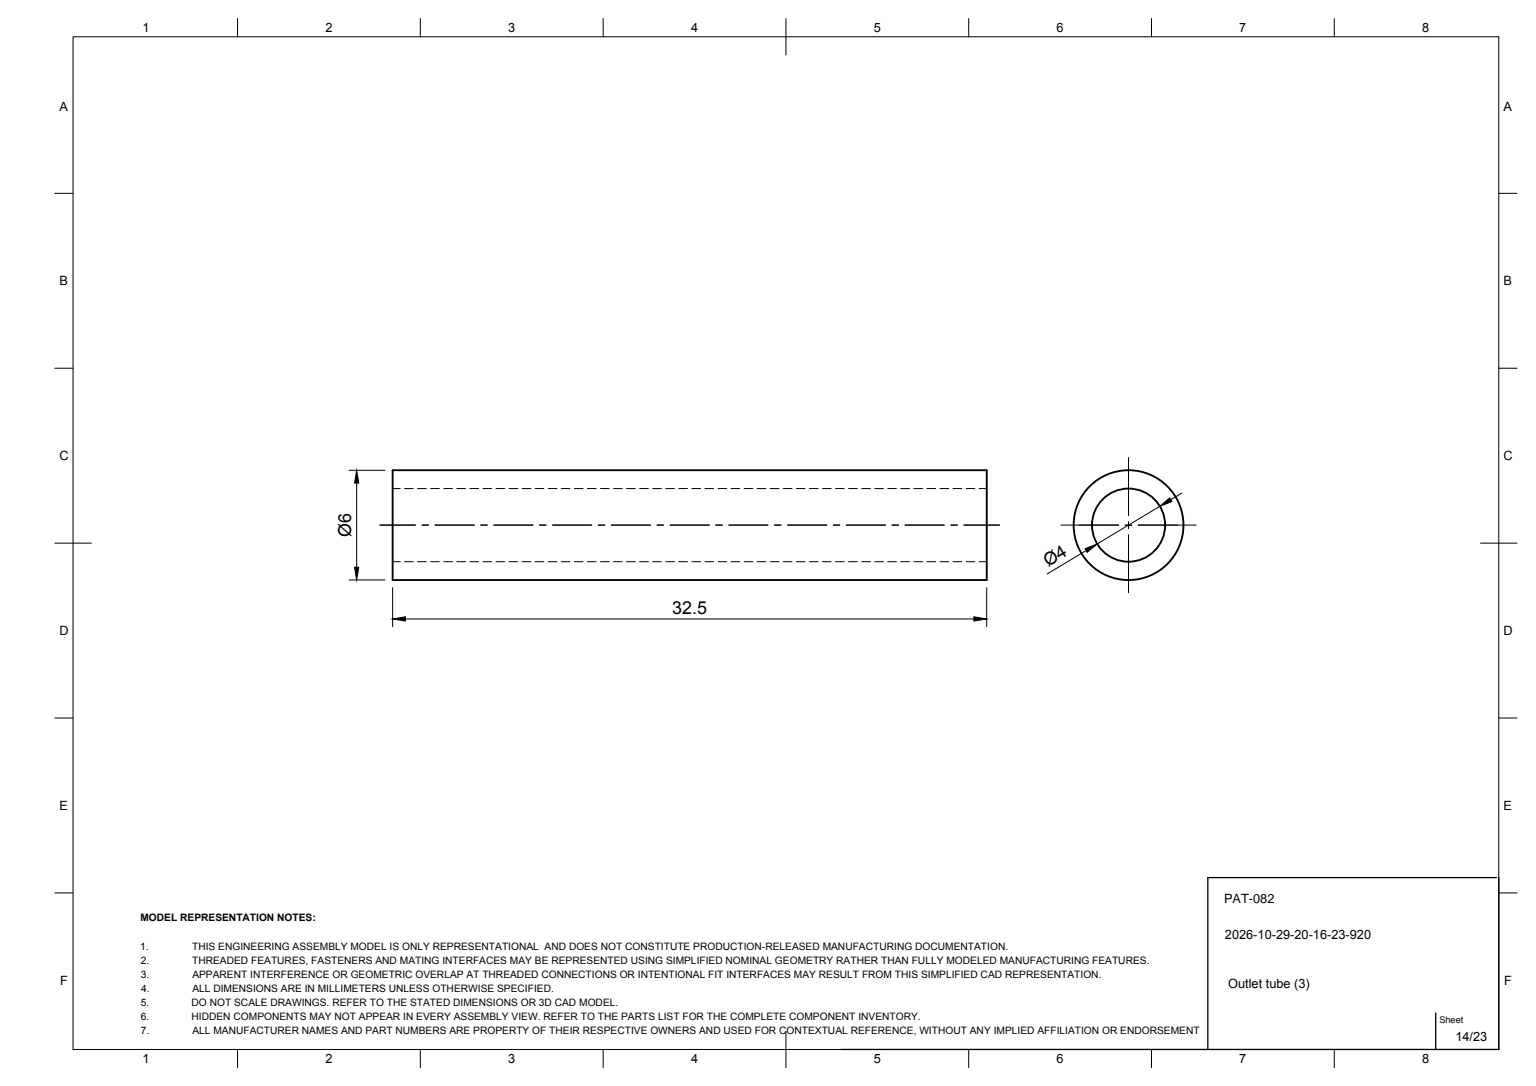
ISO-10303-21;
HEADER;
/* Generated by software containing ST-Developer
 * from STEP Tools, Inc. (www.steptools.com) 
 */

FILE_DESCRIPTION(
/* description */ ('PAT-082'),
/* implementation_level */ '2;1');

FILE_NAME(
/* name */ 'Outlet tube (3).step',
/* time_stamp */ '2026-10-29T20:16:13-07:00',
/* author */ (''),
/* organization */ (''),
/* preprocessor_version */ 'ST-DEVELOPER v20.2',
/* originating_system */ 'Autodesk Translation Framework v15.17.0.0',
/* authorisation */ '');

FILE_SCHEMA (('AUTOMOTIVE_DESIGN { 1 0 10303 214 3 1 1 }'));
ENDSEC;

DATA;
#10=MECHANICAL_DESIGN_GEOMETRIC_PRESENTATION_REPRESENTATION('',(#252),#8266);
#208=SHAPE_REPRESENTATION_RELATIONSHIP('SRR','None',#8370,#230);
#230=ADVANCED_BREP_SHAPE_REPRESENTATION('',(#274),#8254);
#252=STYLED_ITEM('',(#8530),#274);
#274=MANIFOLD_SOLID_BREP('Body1',#4592);
#382=FACE_BOUND('',#1100,.T.);
#383=FACE_BOUND('',#1102,.T.);
#493=PLANE('',#5163);
#494=PLANE('',#5164);
#727=FACE_OUTER_BOUND('',#1097,.T.);
#728=FACE_OUTER_BOUND('',#1098,.T.);
#729=FACE_OUTER_BOUND('',#1099,.T.);
#730=FACE_OUTER_BOUND('',#1101,.T.);
#1097=EDGE_LOOP('',(#3788,#3789,#3790,#3791));
#1098=EDGE_LOOP('',(#3792,#3793,#3794,#3795));
#1099=EDGE_LOOP('',(#3796));
#1100=EDGE_LOOP('',(#3797));
#1101=EDGE_LOOP('',(#3798));
#1102=EDGE_LOOP('',(#3799));
#1434=LINE('',#7700,#1789);
#1435=LINE('',#7706,#1790);
#1789=VECTOR('',#6201,0.2);
#1790=VECTOR('',#6208,0.3);
#2085=CIRCLE('',#5158,0.2);
#2086=CIRCLE('',#5159,0.2);
#2087=CIRCLE('',#5161,0.3);
#2088=CIRCLE('',#5162,0.3);
#2379=VERTEX_POINT('',#7697);
#2380=VERTEX_POINT('',#7699);
#2381=VERTEX_POINT('',#7703);
#2382=VERTEX_POINT('',#7705);
#2870=EDGE_CURVE('',#2379,#2379,#2085,.T.);
#2871=EDGE_CURVE('',#2379,#2380,#1434,.T.);
#2872=EDGE_CURVE('',#2380,#2380,#2086,.T.);
#2873=EDGE_CURVE('',#2381,#2381,#2087,.T.);
#2874=EDGE_CURVE('',#2381,#2382,#1435,.T.);
#2875=EDGE_CURVE('',#2382,#2382,#2088,.T.);
#3788=ORIENTED_EDGE('',*,*,#2870,.F.);
#3789=ORIENTED_EDGE('',*,*,#2871,.T.);
#3790=ORIENTED_EDGE('',*,*,#2872,.T.);
#3791=ORIENTED_EDGE('',*,*,#2871,.F.);
#3792=ORIENTED_EDGE('',*,*,#2873,.F.);
#3793=ORIENTED_EDGE('',*,*,#2874,.T.);
#3794=ORIENTED_EDGE('',*,*,#2875,.T.);
#3795=ORIENTED_EDGE('',*,*,#2874,.F.);
#3796=ORIENTED_EDGE('',*,*,#2873,.T.);
#3797=ORIENTED_EDGE('',*,*,#2870,.T.);
#3798=ORIENTED_EDGE('',*,*,#2875,.F.);
#3799=ORIENTED_EDGE('',*,*,#2872,.F.);
#4287=CYLINDRICAL_SURFACE('',#5157,0.2);
#4288=CYLINDRICAL_SURFACE('',#5160,0.3);
#4466=ADVANCED_FACE('',(#727),#4287,.F.);
#4467=ADVANCED_FACE('',(#728),#4288,.T.);
#4468=ADVANCED_FACE('',(#729,#382),#493,.T.);
#4469=ADVANCED_FACE('',(#730,#383),#494,.F.);
#4592=CLOSED_SHELL('',(#4466,#4467,#4468,#4469));
#5156=AXIS2_PLACEMENT_3D('',#7695,#6195,#6196);
#5157=AXIS2_PLACEMENT_3D('',#7696,#6197,#6198);
#5158=AXIS2_PLACEMENT_3D('',#7698,#6199,#6200);
#5159=AXIS2_PLACEMENT_3D('',#7701,#6202,#6203);
#5160=AXIS2_PLACEMENT_3D('',#7702,#6204,#6205);
#5161=AXIS2_PLACEMENT_3D('',#7704,#6206,#6207);
#5162=AXIS2_PLACEMENT_3D('',#7707,#6209,#6210);
#5163=AXIS2_PLACEMENT_3D('',#7708,#6211,#6212);
#5164=AXIS2_PLACEMENT_3D('',#7709,#6213,#6214);
#6195=DIRECTION('axis',(0.,0.,1.));
#6196=DIRECTION('refdir',(1.,0.,0.));
#6197=DIRECTION('center_axis',(0.,0.,1.));
#6198=DIRECTION('ref_axis',(1.,0.,0.));
#6199=DIRECTION('center_axis',(0.,0.,-1.));
#6200=DIRECTION('ref_axis',(1.,0.,0.));
#6201=DIRECTION('',(0.,0.,-1.));
#6202=DIRECTION('center_axis',(0.,0.,-1.));
#6203=DIRECTION('ref_axis',(1.,0.,0.));
#6204=DIRECTION('center_axis',(0.,0.,1.));
#6205=DIRECTION('ref_axis',(1.,0.,0.));
#6206=DIRECTION('center_axis',(0.,0.,1.));
#6207=DIRECTION('ref_axis',(1.,0.,0.));
#6208=DIRECTION('',(0.,0.,-1.));
#6209=DIRECTION('center_axis',(0.,0.,1.));
#6210=DIRECTION('ref_axis',(1.,0.,0.));
#6211=DIRECTION('center_axis',(0.,0.,1.));
#6212=DIRECTION('ref_axis',(1.,0.,0.));
#6213=DIRECTION('center_axis',(0.,0.,1.));
#6214=DIRECTION('ref_axis',(1.,0.,0.));
#7695=CARTESIAN_POINT('',(0.,0.,0.));
#7696=CARTESIAN_POINT('Origin',(3.75,0.,5.7));
#7697=CARTESIAN_POINT('',(3.55,-2.44929359829471E-17,8.95));
#7698=CARTESIAN_POINT('Origin',(3.75,0.,8.95));
#7699=CARTESIAN_POINT('',(3.55,-2.44929359829471E-17,5.7));
#7700=CARTESIAN_POINT('',(3.55,-2.44929359829471E-17,5.7));
#7701=CARTESIAN_POINT('Origin',(3.75,0.,5.7));
#7702=CARTESIAN_POINT('Origin',(3.75,0.,5.7));
#7703=CARTESIAN_POINT('',(3.45,-3.67394039744206E-17,8.95));
#7704=CARTESIAN_POINT('Origin',(3.75,0.,8.95));
#7705=CARTESIAN_POINT('',(3.45,-3.67394039744206E-17,5.7));
#7706=CARTESIAN_POINT('',(3.45,-3.67394039744206E-17,5.7));
#7707=CARTESIAN_POINT('Origin',(3.75,0.,5.7));
#7708=CARTESIAN_POINT('Origin',(3.75,0.,8.95));
#7709=CARTESIAN_POINT('Origin',(3.75,0.,5.7));
#8229=UNCERTAINTY_MEASURE_WITH_UNIT(LENGTH_MEASURE(0.001),#8267,
'DISTANCE_ACCURACY_VALUE',
'Maximum model space distance between geometric entities at asserted c
onnectivities');
#8241=UNCERTAINTY_MEASURE_WITH_UNIT(LENGTH_MEASURE(0.001),#8267,
'DISTANCE_ACCURACY_VALUE',
'Maximum model space distance between geometric entities at asserted c
onnectivities');
#8254=(
GEOMETRIC_REPRESENTATION_CONTEXT(3)
GLOBAL_UNCERTAINTY_ASSIGNED_CONTEXT((#8229))
GLOBAL_UNIT_ASSIGNED_CONTEXT((#8267,#8269,#8270))
REPRESENTATION_CONTEXT('','3D')
);
#8266=(
GEOMETRIC_REPRESENTATION_CONTEXT(3)
GLOBAL_UNCERTAINTY_ASSIGNED_CONTEXT((#8241))
GLOBAL_UNIT_ASSIGNED_CONTEXT((#8267,#8269,#8270))
REPRESENTATION_CONTEXT('','3D')
);
#8267=(
LENGTH_UNIT()
NAMED_UNIT(*)
SI_UNIT(.CENTI.,.METRE.)
);
#8269=(
NAMED_UNIT(*)
PLANE_ANGLE_UNIT()
SI_UNIT($,.RADIAN.)
);
#8270=(
NAMED_UNIT(*)
SI_UNIT($,.STERADIAN.)
SOLID_ANGLE_UNIT()
);
#8283=SHAPE_DEFINITION_REPRESENTATION(#8307,#8370);
#8307=PRODUCT_DEFINITION_SHAPE('',$,#8395);
#8370=SHAPE_REPRESENTATION('',(#5156),#8254);
#8382=PRODUCT_DEFINITION_CONTEXT('part definition',#8456,'design');
#8395=PRODUCT_DEFINITION('Outlet tube (3)','Outlet tube (3)',
#8419,#8382);
#8419=PRODUCT_DEFINITION_FORMATION('',$,#8470);
#8456=APPLICATION_CONTEXT(
'Core Data for Automotive Mechanical Design Process');
#8457=PRODUCT_CONTEXT('part definition',#8456,'mechanical');
#8470=PRODUCT('Outlet tube (3)','Outlet tube (3)',
'Outlet tube (3)',(#8457));
#8524=COLOUR_RGB('Sky Blue',0.24,0.69,0.87);
#8525=FILL_AREA_STYLE_COLOUR('',#8524);
#8526=FILL_AREA_STYLE('',(#8525));
#8527=SURFACE_STYLE_FILL_AREA(#8526);
#8528=SURFACE_SIDE_STYLE('',(#8527));
#8529=SURFACE_STYLE_USAGE(.BOTH.,#8528);
#8530=PRESENTATION_STYLE_ASSIGNMENT((#8529));
ENDSEC;
END-ISO-10303-21;
